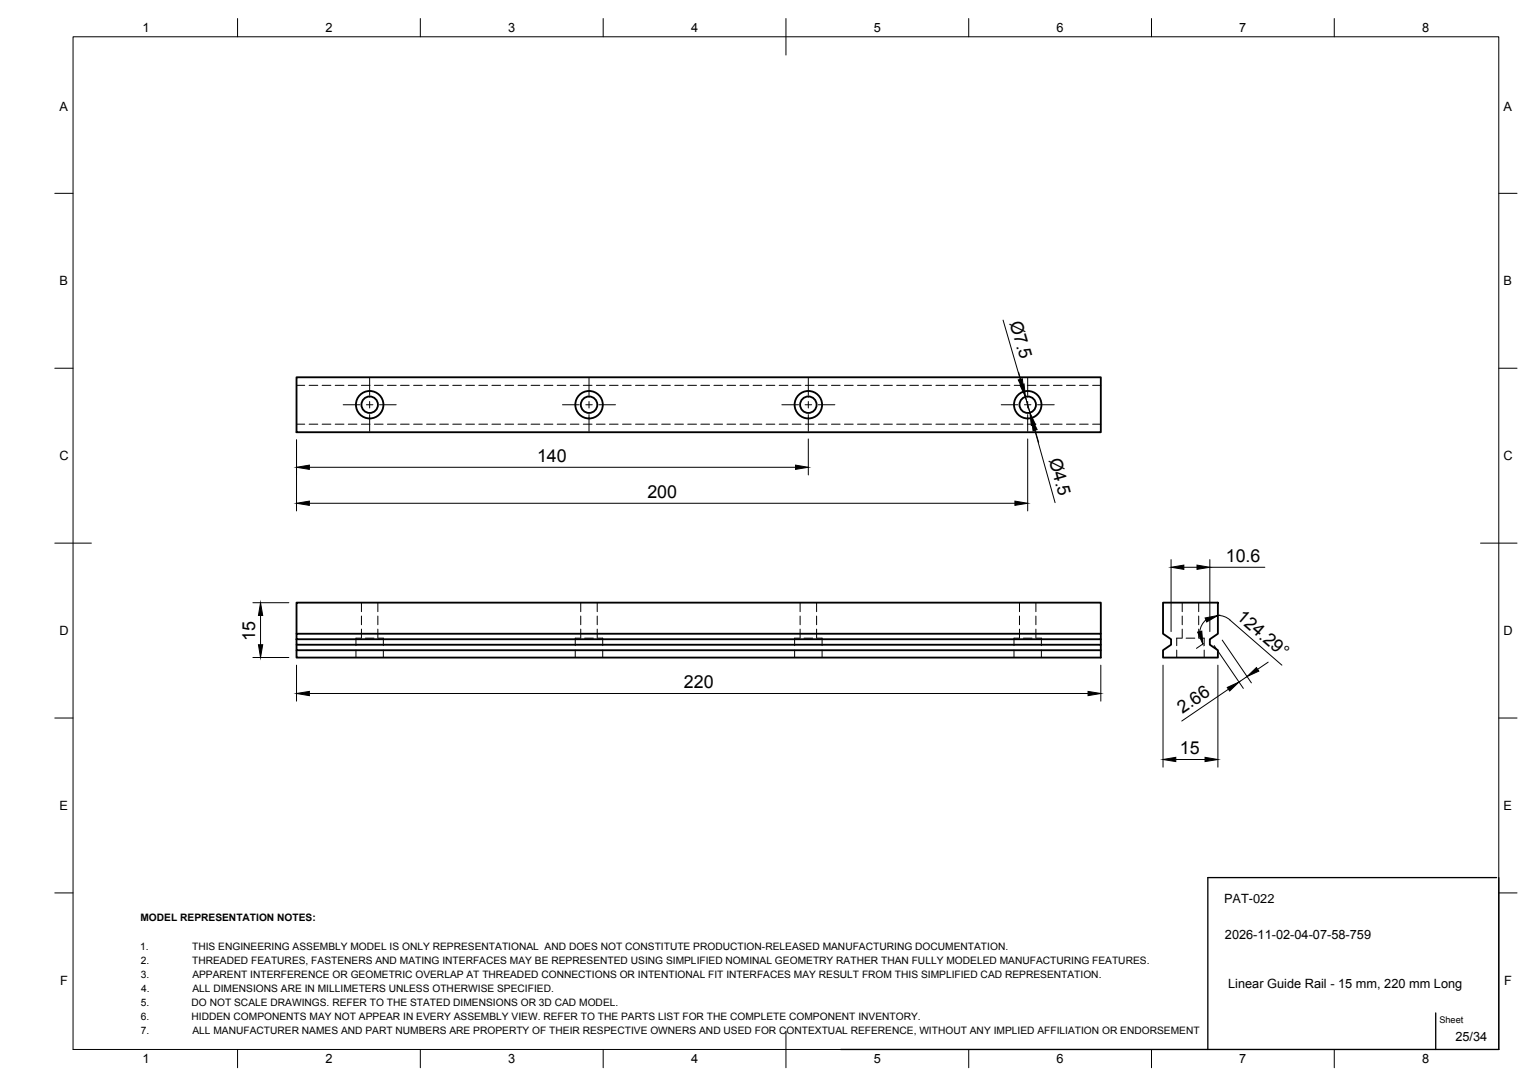
ISO-10303-21;
HEADER;
/* Generated by software containing ST-Developer
 * from STEP Tools, Inc. (www.steptools.com) 
 */

FILE_DESCRIPTION(
/* description */ ('Chute with adjustable gate'),
/* implementation_level */ '2;1');

FILE_NAME(
/* name */ 'Linear Guide Rail - 15 mm, 220 mm Long.step',
/* time_stamp */ '2026-10-27T10:52:28-07:00',
/* author */ (''),
/* organization */ (''),
/* preprocessor_version */ 'ST-DEVELOPER v20.2',
/* originating_system */ 'Autodesk Translation Framework v15.17.0.0',
/* authorisation */ '');

FILE_SCHEMA (('AUTOMOTIVE_DESIGN { 1 0 10303 214 3 1 1 }'));
ENDSEC;

DATA;
#10=MECHANICAL_DESIGN_GEOMETRIC_PRESENTATION_REPRESENTATION('',(#435),#13094);
#371=SHAPE_REPRESENTATION_RELATIONSHIP('SRR','None',#13272,#403);
#403=ADVANCED_BREP_SHAPE_REPRESENTATION('',(#466),#13081);
#435=STYLED_ITEM('',(#13488),#466);
#466=MANIFOLD_SOLID_BREP('Body1',#7619);
#553=FACE_BOUND('',#1658,.T.);
#554=FACE_BOUND('',#1661,.T.);
#555=FACE_BOUND('',#1664,.T.);
#556=FACE_BOUND('',#1667,.T.);
#557=FACE_BOUND('',#1677,.T.);
#558=FACE_BOUND('',#1678,.T.);
#559=FACE_BOUND('',#1679,.T.);
#560=FACE_BOUND('',#1680,.T.);
#561=FACE_BOUND('',#1687,.T.);
#562=FACE_BOUND('',#1688,.T.);
#563=FACE_BOUND('',#1689,.T.);
#564=FACE_BOUND('',#1690,.T.);
#791=PLANE('',#8351);
#792=PLANE('',#8356);
#793=PLANE('',#8361);
#794=PLANE('',#8366);
#795=PLANE('',#8376);
#796=PLANE('',#8377);
#797=PLANE('',#8378);
#798=PLANE('',#8379);
#799=PLANE('',#8380);
#800=PLANE('',#8381);
#801=PLANE('',#8382);
#802=PLANE('',#8383);
#803=PLANE('',#8384);
#804=PLANE('',#8385);
#805=PLANE('',#8386);
#806=PLANE('',#8387);
#807=PLANE('',#8388);
#808=PLANE('',#8389);
#1162=FACE_OUTER_BOUND('',#1656,.T.);
#1163=FACE_OUTER_BOUND('',#1657,.T.);
#1164=FACE_OUTER_BOUND('',#1659,.T.);
#1165=FACE_OUTER_BOUND('',#1660,.T.);
#1166=FACE_OUTER_BOUND('',#1662,.T.);
#1167=FACE_OUTER_BOUND('',#1663,.T.);
#1168=FACE_OUTER_BOUND('',#1665,.T.);
#1169=FACE_OUTER_BOUND('',#1666,.T.);
#1170=FACE_OUTER_BOUND('',#1668,.T.);
#1171=FACE_OUTER_BOUND('',#1669,.T.);
#1172=FACE_OUTER_BOUND('',#1670,.T.);
#1173=FACE_OUTER_BOUND('',#1671,.T.);
#1174=FACE_OUTER_BOUND('',#1672,.T.);
#1175=FACE_OUTER_BOUND('',#1673,.T.);
#1176=FACE_OUTER_BOUND('',#1674,.T.);
#1177=FACE_OUTER_BOUND('',#1675,.T.);
#1178=FACE_OUTER_BOUND('',#1676,.T.);
#1179=FACE_OUTER_BOUND('',#1681,.T.);
#1180=FACE_OUTER_BOUND('',#1682,.T.);
#1181=FACE_OUTER_BOUND('',#1683,.T.);
#1182=FACE_OUTER_BOUND('',#1684,.T.);
#1183=FACE_OUTER_BOUND('',#1685,.T.);
#1184=FACE_OUTER_BOUND('',#1686,.T.);
#1185=FACE_OUTER_BOUND('',#1691,.T.);
#1186=FACE_OUTER_BOUND('',#1692,.T.);
#1187=FACE_OUTER_BOUND('',#1693,.T.);
#1656=EDGE_LOOP('',(#6336,#6337,#6338,#6339));
#1657=EDGE_LOOP('',(#6340));
#1658=EDGE_LOOP('',(#6341));
#1659=EDGE_LOOP('',(#6342,#6343,#6344,#6345));
#1660=EDGE_LOOP('',(#6346));
#1661=EDGE_LOOP('',(#6347));
#1662=EDGE_LOOP('',(#6348,#6349,#6350,#6351));
#1663=EDGE_LOOP('',(#6352));
#1664=EDGE_LOOP('',(#6353));
#1665=EDGE_LOOP('',(#6354,#6355,#6356,#6357));
#1666=EDGE_LOOP('',(#6358));
#1667=EDGE_LOOP('',(#6359));
#1668=EDGE_LOOP('',(#6360,#6361,#6362,#6363));
#1669=EDGE_LOOP('',(#6364,#6365,#6366,#6367));
#1670=EDGE_LOOP('',(#6368,#6369,#6370,#6371));
#1671=EDGE_LOOP('',(#6372,#6373,#6374,#6375));
#1672=EDGE_LOOP('',(#6376,#6377,#6378,#6379));
#1673=EDGE_LOOP('',(#6380,#6381,#6382,#6383));
#1674=EDGE_LOOP('',(#6384,#6385,#6386,#6387));
#1675=EDGE_LOOP('',(#6388,#6389,#6390,#6391));
#1676=EDGE_LOOP('',(#6392,#6393,#6394,#6395));
#1677=EDGE_LOOP('',(#6396));
#1678=EDGE_LOOP('',(#6397));
#1679=EDGE_LOOP('',(#6398));
#1680=EDGE_LOOP('',(#6399));
#1681=EDGE_LOOP('',(#6400,#6401,#6402,#6403));
#1682=EDGE_LOOP('',(#6404,#6405,#6406,#6407));
#1683=EDGE_LOOP('',(#6408,#6409,#6410,#6411));
#1684=EDGE_LOOP('',(#6412,#6413,#6414,#6415));
#1685=EDGE_LOOP('',(#6416,#6417,#6418,#6419));
#1686=EDGE_LOOP('',(#6420,#6421,#6422,#6423));
#1687=EDGE_LOOP('',(#6424));
#1688=EDGE_LOOP('',(#6425));
#1689=EDGE_LOOP('',(#6426));
#1690=EDGE_LOOP('',(#6427));
#1691=EDGE_LOOP('',(#6428,#6429,#6430,#6431));
#1692=EDGE_LOOP('',(#6432,#6433,#6434,#6435,#6436,#6437,#6438,#6439,#6440,
#6441,#6442,#6443));
#1693=EDGE_LOOP('',(#6444,#6445,#6446,#6447,#6448,#6449,#6450,#6451,#6452,
#6453,#6454,#6455));
#2345=LINE('',#12132,#3122);
#2346=LINE('',#12141,#3123);
#2347=LINE('',#12150,#3124);
#2348=LINE('',#12159,#3125);
#2349=LINE('',#12167,#3126);
#2350=LINE('',#12171,#3127);
#2351=LINE('',#12175,#3128);
#2352=LINE('',#12179,#3129);
#2353=LINE('',#12183,#3130);
#2354=LINE('',#12185,#3131);
#2355=LINE('',#12187,#3132);
#2356=LINE('',#12188,#3133);
#2357=LINE('',#12191,#3134);
#2358=LINE('',#12193,#3135);
#2359=LINE('',#12194,#3136);
#2360=LINE('',#12197,#3137);
#2361=LINE('',#12199,#3138);
#2362=LINE('',#12200,#3139);
#2363=LINE('',#12203,#3140);
#2364=LINE('',#12205,#3141);
#2365=LINE('',#12206,#3142);
#2366=LINE('',#12209,#3143);
#2367=LINE('',#12211,#3144);
#2368=LINE('',#12212,#3145);
#2369=LINE('',#12215,#3146);
#2370=LINE('',#12217,#3147);
#2371=LINE('',#12218,#3148);
#2372=LINE('',#12221,#3149);
#2373=LINE('',#12223,#3150);
#2374=LINE('',#12224,#3151);
#2375=LINE('',#12227,#3152);
#2376=LINE('',#12229,#3153);
#2377=LINE('',#12230,#3154);
#2378=LINE('',#12233,#3155);
#2379=LINE('',#12235,#3156);
#2380=LINE('',#12236,#3157);
#2381=LINE('',#12239,#3158);
#2382=LINE('',#12241,#3159);
#2383=LINE('',#12242,#3160);
#2384=LINE('',#12245,#3161);
#2385=LINE('',#12247,#3162);
#2386=LINE('',#12248,#3163);
#2387=LINE('',#12250,#3164);
#2388=LINE('',#12251,#3165);
#3122=VECTOR('',#9911,0.375);
#3123=VECTOR('',#9922,0.375);
#3124=VECTOR('',#9933,0.375);
#3125=VECTOR('',#9944,0.375);
#3126=VECTOR('',#9955,0.225);
#3127=VECTOR('',#9960,0.225);
#3128=VECTOR('',#9965,0.225);
#3129=VECTOR('',#9970,0.225000000000001);
#3130=VECTOR('',#9973,1.);
#3131=VECTOR('',#9974,1.);
#3132=VECTOR('',#9975,1.);
#3133=VECTOR('',#9976,1.);
#3134=VECTOR('',#9979,1.);
#3135=VECTOR('',#9980,1.);
#3136=VECTOR('',#9981,1.);
#3137=VECTOR('',#9984,1.);
#3138=VECTOR('',#9985,1.);
#3139=VECTOR('',#9986,1.);
#3140=VECTOR('',#9989,1.);
#3141=VECTOR('',#9990,1.);
#3142=VECTOR('',#9991,1.);
#3143=VECTOR('',#9994,1.);
#3144=VECTOR('',#9995,1.);
#3145=VECTOR('',#9996,1.);
#3146=VECTOR('',#9999,1.);
#3147=VECTOR('',#10000,1.);
#3148=VECTOR('',#10001,1.);
#3149=VECTOR('',#10004,1.);
#3150=VECTOR('',#10005,1.);
#3151=VECTOR('',#10006,1.);
#3152=VECTOR('',#10009,1.);
#3153=VECTOR('',#10010,1.);
#3154=VECTOR('',#10011,1.);
#3155=VECTOR('',#10014,1.);
#3156=VECTOR('',#10015,1.);
#3157=VECTOR('',#10016,1.);
#3158=VECTOR('',#10019,1.);
#3159=VECTOR('',#10020,1.);
#3160=VECTOR('',#10021,1.);
#3161=VECTOR('',#10024,1.);
#3162=VECTOR('',#10025,1.);
#3163=VECTOR('',#10026,1.);
#3164=VECTOR('',#10029,1.);
#3165=VECTOR('',#10030,1.);
#3504=CIRCLE('',#8349,0.375);
#3505=CIRCLE('',#8350,0.375);
#3506=CIRCLE('',#8352,0.225);
#3507=CIRCLE('',#8354,0.375);
#3508=CIRCLE('',#8355,0.375);
#3509=CIRCLE('',#8357,0.225);
#3510=CIRCLE('',#8359,0.375);
#3511=CIRCLE('',#8360,0.375);
#3512=CIRCLE('',#8362,0.225);
#3513=CIRCLE('',#8364,0.375);
#3514=CIRCLE('',#8365,0.375);
#3515=CIRCLE('',#8367,0.225000000000001);
#3516=CIRCLE('',#8369,0.225);
#3517=CIRCLE('',#8371,0.225);
#3518=CIRCLE('',#8373,0.225);
#3519=CIRCLE('',#8375,0.225000000000001);
#3975=VERTEX_POINT('',#12129);
#3976=VERTEX_POINT('',#12131);
#3977=VERTEX_POINT('',#12135);
#3978=VERTEX_POINT('',#12138);
#3979=VERTEX_POINT('',#12140);
#3980=VERTEX_POINT('',#12144);
#3981=VERTEX_POINT('',#12147);
#3982=VERTEX_POINT('',#12149);
#3983=VERTEX_POINT('',#12153);
#3984=VERTEX_POINT('',#12156);
#3985=VERTEX_POINT('',#12158);
#3986=VERTEX_POINT('',#12162);
#3987=VERTEX_POINT('',#12165);
#3988=VERTEX_POINT('',#12169);
#3989=VERTEX_POINT('',#12173);
#3990=VERTEX_POINT('',#12177);
#3991=VERTEX_POINT('',#12181);
#3992=VERTEX_POINT('',#12182);
#3993=VERTEX_POINT('',#12184);
#3994=VERTEX_POINT('',#12186);
#3995=VERTEX_POINT('',#12190);
#3996=VERTEX_POINT('',#12192);
#3997=VERTEX_POINT('',#12196);
#3998=VERTEX_POINT('',#12198);
#3999=VERTEX_POINT('',#12202);
#4000=VERTEX_POINT('',#12204);
#4001=VERTEX_POINT('',#12208);
#4002=VERTEX_POINT('',#12210);
#4003=VERTEX_POINT('',#12214);
#4004=VERTEX_POINT('',#12216);
#4005=VERTEX_POINT('',#12220);
#4006=VERTEX_POINT('',#12222);
#4007=VERTEX_POINT('',#12226);
#4008=VERTEX_POINT('',#12228);
#4009=VERTEX_POINT('',#12232);
#4010=VERTEX_POINT('',#12234);
#4011=VERTEX_POINT('',#12238);
#4012=VERTEX_POINT('',#12240);
#4013=VERTEX_POINT('',#12244);
#4014=VERTEX_POINT('',#12246);
#4801=EDGE_CURVE('',#3975,#3975,#3504,.T.);
#4802=EDGE_CURVE('',#3975,#3976,#2345,.T.);
#4803=EDGE_CURVE('',#3976,#3976,#3505,.T.);
#4804=EDGE_CURVE('',#3977,#3977,#3506,.T.);
#4805=EDGE_CURVE('',#3978,#3978,#3507,.T.);
#4806=EDGE_CURVE('',#3978,#3979,#2346,.T.);
#4807=EDGE_CURVE('',#3979,#3979,#3508,.T.);
#4808=EDGE_CURVE('',#3980,#3980,#3509,.T.);
#4809=EDGE_CURVE('',#3981,#3981,#3510,.T.);
#4810=EDGE_CURVE('',#3981,#3982,#2347,.T.);
#4811=EDGE_CURVE('',#3982,#3982,#3511,.T.);
#4812=EDGE_CURVE('',#3983,#3983,#3512,.T.);
#4813=EDGE_CURVE('',#3984,#3984,#3513,.T.);
#4814=EDGE_CURVE('',#3984,#3985,#2348,.T.);
#4815=EDGE_CURVE('',#3985,#3985,#3514,.T.);
#4816=EDGE_CURVE('',#3986,#3986,#3515,.T.);
#4817=EDGE_CURVE('',#3987,#3987,#3516,.T.);
#4818=EDGE_CURVE('',#3987,#3977,#2349,.T.);
#4819=EDGE_CURVE('',#3988,#3988,#3517,.T.);
#4820=EDGE_CURVE('',#3988,#3980,#2350,.T.);
#4821=EDGE_CURVE('',#3989,#3989,#3518,.T.);
#4822=EDGE_CURVE('',#3989,#3983,#2351,.T.);
#4823=EDGE_CURVE('',#3990,#3990,#3519,.T.);
#4824=EDGE_CURVE('',#3990,#3986,#2352,.T.);
#4825=EDGE_CURVE('',#3991,#3992,#2353,.T.);
#4826=EDGE_CURVE('',#3992,#3993,#2354,.T.);
#4827=EDGE_CURVE('',#3994,#3993,#2355,.T.);
#4828=EDGE_CURVE('',#3991,#3994,#2356,.T.);
#4829=EDGE_CURVE('',#3995,#3991,#2357,.T.);
#4830=EDGE_CURVE('',#3996,#3994,#2358,.T.);
#4831=EDGE_CURVE('',#3995,#3996,#2359,.T.);
#4832=EDGE_CURVE('',#3997,#3995,#2360,.T.);
#4833=EDGE_CURVE('',#3998,#3996,#2361,.T.);
#4834=EDGE_CURVE('',#3997,#3998,#2362,.T.);
#4835=EDGE_CURVE('',#3999,#3997,#2363,.T.);
#4836=EDGE_CURVE('',#4000,#3998,#2364,.T.);
#4837=EDGE_CURVE('',#3999,#4000,#2365,.T.);
#4838=EDGE_CURVE('',#4001,#3999,#2366,.T.);
#4839=EDGE_CURVE('',#4002,#4000,#2367,.T.);
#4840=EDGE_CURVE('',#4001,#4002,#2368,.T.);
#4841=EDGE_CURVE('',#4003,#4001,#2369,.T.);
#4842=EDGE_CURVE('',#4004,#4002,#2370,.T.);
#4843=EDGE_CURVE('',#4003,#4004,#2371,.T.);
#4844=EDGE_CURVE('',#4005,#4003,#2372,.T.);
#4845=EDGE_CURVE('',#4006,#4004,#2373,.T.);
#4846=EDGE_CURVE('',#4005,#4006,#2374,.T.);
#4847=EDGE_CURVE('',#4007,#4005,#2375,.T.);
#4848=EDGE_CURVE('',#4008,#4006,#2376,.T.);
#4849=EDGE_CURVE('',#4007,#4008,#2377,.T.);
#4850=EDGE_CURVE('',#4009,#4007,#2378,.T.);
#4851=EDGE_CURVE('',#4010,#4008,#2379,.T.);
#4852=EDGE_CURVE('',#4009,#4010,#2380,.T.);
#4853=EDGE_CURVE('',#4011,#4009,#2381,.T.);
#4854=EDGE_CURVE('',#4012,#4010,#2382,.T.);
#4855=EDGE_CURVE('',#4011,#4012,#2383,.T.);
#4856=EDGE_CURVE('',#4013,#4011,#2384,.T.);
#4857=EDGE_CURVE('',#4014,#4012,#2385,.T.);
#4858=EDGE_CURVE('',#4013,#4014,#2386,.T.);
#4859=EDGE_CURVE('',#3992,#4013,#2387,.T.);
#4860=EDGE_CURVE('',#3993,#4014,#2388,.T.);
#6336=ORIENTED_EDGE('',*,*,#4801,.F.);
#6337=ORIENTED_EDGE('',*,*,#4802,.T.);
#6338=ORIENTED_EDGE('',*,*,#4803,.F.);
#6339=ORIENTED_EDGE('',*,*,#4802,.F.);
#6340=ORIENTED_EDGE('',*,*,#4801,.T.);
#6341=ORIENTED_EDGE('',*,*,#4804,.F.);
#6342=ORIENTED_EDGE('',*,*,#4805,.F.);
#6343=ORIENTED_EDGE('',*,*,#4806,.T.);
#6344=ORIENTED_EDGE('',*,*,#4807,.F.);
#6345=ORIENTED_EDGE('',*,*,#4806,.F.);
#6346=ORIENTED_EDGE('',*,*,#4805,.T.);
#6347=ORIENTED_EDGE('',*,*,#4808,.F.);
#6348=ORIENTED_EDGE('',*,*,#4809,.F.);
#6349=ORIENTED_EDGE('',*,*,#4810,.T.);
#6350=ORIENTED_EDGE('',*,*,#4811,.F.);
#6351=ORIENTED_EDGE('',*,*,#4810,.F.);
#6352=ORIENTED_EDGE('',*,*,#4809,.T.);
#6353=ORIENTED_EDGE('',*,*,#4812,.F.);
#6354=ORIENTED_EDGE('',*,*,#4813,.F.);
#6355=ORIENTED_EDGE('',*,*,#4814,.T.);
#6356=ORIENTED_EDGE('',*,*,#4815,.F.);
#6357=ORIENTED_EDGE('',*,*,#4814,.F.);
#6358=ORIENTED_EDGE('',*,*,#4813,.T.);
#6359=ORIENTED_EDGE('',*,*,#4816,.F.);
#6360=ORIENTED_EDGE('',*,*,#4817,.F.);
#6361=ORIENTED_EDGE('',*,*,#4818,.T.);
#6362=ORIENTED_EDGE('',*,*,#4804,.T.);
#6363=ORIENTED_EDGE('',*,*,#4818,.F.);
#6364=ORIENTED_EDGE('',*,*,#4819,.F.);
#6365=ORIENTED_EDGE('',*,*,#4820,.T.);
#6366=ORIENTED_EDGE('',*,*,#4808,.T.);
#6367=ORIENTED_EDGE('',*,*,#4820,.F.);
#6368=ORIENTED_EDGE('',*,*,#4821,.F.);
#6369=ORIENTED_EDGE('',*,*,#4822,.T.);
#6370=ORIENTED_EDGE('',*,*,#4812,.T.);
#6371=ORIENTED_EDGE('',*,*,#4822,.F.);
#6372=ORIENTED_EDGE('',*,*,#4823,.F.);
#6373=ORIENTED_EDGE('',*,*,#4824,.T.);
#6374=ORIENTED_EDGE('',*,*,#4816,.T.);
#6375=ORIENTED_EDGE('',*,*,#4824,.F.);
#6376=ORIENTED_EDGE('',*,*,#4825,.T.);
#6377=ORIENTED_EDGE('',*,*,#4826,.T.);
#6378=ORIENTED_EDGE('',*,*,#4827,.F.);
#6379=ORIENTED_EDGE('',*,*,#4828,.F.);
#6380=ORIENTED_EDGE('',*,*,#4829,.T.);
#6381=ORIENTED_EDGE('',*,*,#4828,.T.);
#6382=ORIENTED_EDGE('',*,*,#4830,.F.);
#6383=ORIENTED_EDGE('',*,*,#4831,.F.);
#6384=ORIENTED_EDGE('',*,*,#4832,.T.);
#6385=ORIENTED_EDGE('',*,*,#4831,.T.);
#6386=ORIENTED_EDGE('',*,*,#4833,.F.);
#6387=ORIENTED_EDGE('',*,*,#4834,.F.);
#6388=ORIENTED_EDGE('',*,*,#4835,.T.);
#6389=ORIENTED_EDGE('',*,*,#4834,.T.);
#6390=ORIENTED_EDGE('',*,*,#4836,.F.);
#6391=ORIENTED_EDGE('',*,*,#4837,.F.);
#6392=ORIENTED_EDGE('',*,*,#4838,.T.);
#6393=ORIENTED_EDGE('',*,*,#4837,.T.);
#6394=ORIENTED_EDGE('',*,*,#4839,.F.);
#6395=ORIENTED_EDGE('',*,*,#4840,.F.);
#6396=ORIENTED_EDGE('',*,*,#4815,.T.);
#6397=ORIENTED_EDGE('',*,*,#4811,.T.);
#6398=ORIENTED_EDGE('',*,*,#4807,.T.);
#6399=ORIENTED_EDGE('',*,*,#4803,.T.);
#6400=ORIENTED_EDGE('',*,*,#4841,.T.);
#6401=ORIENTED_EDGE('',*,*,#4840,.T.);
#6402=ORIENTED_EDGE('',*,*,#4842,.F.);
#6403=ORIENTED_EDGE('',*,*,#4843,.F.);
#6404=ORIENTED_EDGE('',*,*,#4844,.T.);
#6405=ORIENTED_EDGE('',*,*,#4843,.T.);
#6406=ORIENTED_EDGE('',*,*,#4845,.F.);
#6407=ORIENTED_EDGE('',*,*,#4846,.F.);
#6408=ORIENTED_EDGE('',*,*,#4847,.T.);
#6409=ORIENTED_EDGE('',*,*,#4846,.T.);
#6410=ORIENTED_EDGE('',*,*,#4848,.F.);
#6411=ORIENTED_EDGE('',*,*,#4849,.F.);
#6412=ORIENTED_EDGE('',*,*,#4850,.T.);
#6413=ORIENTED_EDGE('',*,*,#4849,.T.);
#6414=ORIENTED_EDGE('',*,*,#4851,.F.);
#6415=ORIENTED_EDGE('',*,*,#4852,.F.);
#6416=ORIENTED_EDGE('',*,*,#4853,.T.);
#6417=ORIENTED_EDGE('',*,*,#4852,.T.);
#6418=ORIENTED_EDGE('',*,*,#4854,.F.);
#6419=ORIENTED_EDGE('',*,*,#4855,.F.);
#6420=ORIENTED_EDGE('',*,*,#4856,.T.);
#6421=ORIENTED_EDGE('',*,*,#4855,.T.);
#6422=ORIENTED_EDGE('',*,*,#4857,.F.);
#6423=ORIENTED_EDGE('',*,*,#4858,.F.);
#6424=ORIENTED_EDGE('',*,*,#4817,.T.);
#6425=ORIENTED_EDGE('',*,*,#4819,.T.);
#6426=ORIENTED_EDGE('',*,*,#4821,.T.);
#6427=ORIENTED_EDGE('',*,*,#4823,.T.);
#6428=ORIENTED_EDGE('',*,*,#4859,.T.);
#6429=ORIENTED_EDGE('',*,*,#4858,.T.);
#6430=ORIENTED_EDGE('',*,*,#4860,.F.);
#6431=ORIENTED_EDGE('',*,*,#4826,.F.);
#6432=ORIENTED_EDGE('',*,*,#4860,.T.);
#6433=ORIENTED_EDGE('',*,*,#4857,.T.);
#6434=ORIENTED_EDGE('',*,*,#4854,.T.);
#6435=ORIENTED_EDGE('',*,*,#4851,.T.);
#6436=ORIENTED_EDGE('',*,*,#4848,.T.);
#6437=ORIENTED_EDGE('',*,*,#4845,.T.);
#6438=ORIENTED_EDGE('',*,*,#4842,.T.);
#6439=ORIENTED_EDGE('',*,*,#4839,.T.);
#6440=ORIENTED_EDGE('',*,*,#4836,.T.);
#6441=ORIENTED_EDGE('',*,*,#4833,.T.);
#6442=ORIENTED_EDGE('',*,*,#4830,.T.);
#6443=ORIENTED_EDGE('',*,*,#4827,.T.);
#6444=ORIENTED_EDGE('',*,*,#4859,.F.);
#6445=ORIENTED_EDGE('',*,*,#4825,.F.);
#6446=ORIENTED_EDGE('',*,*,#4829,.F.);
#6447=ORIENTED_EDGE('',*,*,#4832,.F.);
#6448=ORIENTED_EDGE('',*,*,#4835,.F.);
#6449=ORIENTED_EDGE('',*,*,#4838,.F.);
#6450=ORIENTED_EDGE('',*,*,#4841,.F.);
#6451=ORIENTED_EDGE('',*,*,#4844,.F.);
#6452=ORIENTED_EDGE('',*,*,#4847,.F.);
#6453=ORIENTED_EDGE('',*,*,#4850,.F.);
#6454=ORIENTED_EDGE('',*,*,#4853,.F.);
#6455=ORIENTED_EDGE('',*,*,#4856,.F.);
#7149=CYLINDRICAL_SURFACE('',#8348,0.375);
#7150=CYLINDRICAL_SURFACE('',#8353,0.375);
#7151=CYLINDRICAL_SURFACE('',#8358,0.375);
#7152=CYLINDRICAL_SURFACE('',#8363,0.375);
#7153=CYLINDRICAL_SURFACE('',#8368,0.225);
#7154=CYLINDRICAL_SURFACE('',#8370,0.225);
#7155=CYLINDRICAL_SURFACE('',#8372,0.225);
#7156=CYLINDRICAL_SURFACE('',#8374,0.225000000000001);
#7430=ADVANCED_FACE('',(#1162),#7149,.F.);
#7431=ADVANCED_FACE('',(#1163,#553),#791,.T.);
#7432=ADVANCED_FACE('',(#1164),#7150,.F.);
#7433=ADVANCED_FACE('',(#1165,#554),#792,.T.);
#7434=ADVANCED_FACE('',(#1166),#7151,.F.);
#7435=ADVANCED_FACE('',(#1167,#555),#793,.T.);
#7436=ADVANCED_FACE('',(#1168),#7152,.F.);
#7437=ADVANCED_FACE('',(#1169,#556),#794,.T.);
#7438=ADVANCED_FACE('',(#1170),#7153,.F.);
#7439=ADVANCED_FACE('',(#1171),#7154,.F.);
#7440=ADVANCED_FACE('',(#1172),#7155,.F.);
#7441=ADVANCED_FACE('',(#1173),#7156,.F.);
#7442=ADVANCED_FACE('',(#1174),#795,.T.);
#7443=ADVANCED_FACE('',(#1175),#796,.T.);
#7444=ADVANCED_FACE('',(#1176),#797,.T.);
#7445=ADVANCED_FACE('',(#1177),#798,.T.);
#7446=ADVANCED_FACE('',(#1178,#557,#558,#559,#560),#799,.T.);
#7447=ADVANCED_FACE('',(#1179),#800,.T.);
#7448=ADVANCED_FACE('',(#1180),#801,.T.);
#7449=ADVANCED_FACE('',(#1181),#802,.T.);
#7450=ADVANCED_FACE('',(#1182),#803,.T.);
#7451=ADVANCED_FACE('',(#1183),#804,.T.);
#7452=ADVANCED_FACE('',(#1184,#561,#562,#563,#564),#805,.T.);
#7453=ADVANCED_FACE('',(#1185),#806,.T.);
#7454=ADVANCED_FACE('',(#1186),#807,.T.);
#7455=ADVANCED_FACE('',(#1187),#808,.F.);
#7619=CLOSED_SHELL('',(#7430,#7431,#7432,#7433,#7434,#7435,#7436,#7437,
#7438,#7439,#7440,#7441,#7442,#7443,#7444,#7445,#7446,#7447,#7448,#7449,
#7450,#7451,#7452,#7453,#7454,#7455));
#8347=AXIS2_PLACEMENT_3D('',#12127,#9905,#9906);
#8348=AXIS2_PLACEMENT_3D('',#12128,#9907,#9908);
#8349=AXIS2_PLACEMENT_3D('',#12130,#9909,#9910);
#8350=AXIS2_PLACEMENT_3D('',#12133,#9912,#9913);
#8351=AXIS2_PLACEMENT_3D('',#12134,#9914,#9915);
#8352=AXIS2_PLACEMENT_3D('',#12136,#9916,#9917);
#8353=AXIS2_PLACEMENT_3D('',#12137,#9918,#9919);
#8354=AXIS2_PLACEMENT_3D('',#12139,#9920,#9921);
#8355=AXIS2_PLACEMENT_3D('',#12142,#9923,#9924);
#8356=AXIS2_PLACEMENT_3D('',#12143,#9925,#9926);
#8357=AXIS2_PLACEMENT_3D('',#12145,#9927,#9928);
#8358=AXIS2_PLACEMENT_3D('',#12146,#9929,#9930);
#8359=AXIS2_PLACEMENT_3D('',#12148,#9931,#9932);
#8360=AXIS2_PLACEMENT_3D('',#12151,#9934,#9935);
#8361=AXIS2_PLACEMENT_3D('',#12152,#9936,#9937);
#8362=AXIS2_PLACEMENT_3D('',#12154,#9938,#9939);
#8363=AXIS2_PLACEMENT_3D('',#12155,#9940,#9941);
#8364=AXIS2_PLACEMENT_3D('',#12157,#9942,#9943);
#8365=AXIS2_PLACEMENT_3D('',#12160,#9945,#9946);
#8366=AXIS2_PLACEMENT_3D('',#12161,#9947,#9948);
#8367=AXIS2_PLACEMENT_3D('',#12163,#9949,#9950);
#8368=AXIS2_PLACEMENT_3D('',#12164,#9951,#9952);
#8369=AXIS2_PLACEMENT_3D('',#12166,#9953,#9954);
#8370=AXIS2_PLACEMENT_3D('',#12168,#9956,#9957);
#8371=AXIS2_PLACEMENT_3D('',#12170,#9958,#9959);
#8372=AXIS2_PLACEMENT_3D('',#12172,#9961,#9962);
#8373=AXIS2_PLACEMENT_3D('',#12174,#9963,#9964);
#8374=AXIS2_PLACEMENT_3D('',#12176,#9966,#9967);
#8375=AXIS2_PLACEMENT_3D('',#12178,#9968,#9969);
#8376=AXIS2_PLACEMENT_3D('',#12180,#9971,#9972);
#8377=AXIS2_PLACEMENT_3D('',#12189,#9977,#9978);
#8378=AXIS2_PLACEMENT_3D('',#12195,#9982,#9983);
#8379=AXIS2_PLACEMENT_3D('',#12201,#9987,#9988);
#8380=AXIS2_PLACEMENT_3D('',#12207,#9992,#9993);
#8381=AXIS2_PLACEMENT_3D('',#12213,#9997,#9998);
#8382=AXIS2_PLACEMENT_3D('',#12219,#10002,#10003);
#8383=AXIS2_PLACEMENT_3D('',#12225,#10007,#10008);
#8384=AXIS2_PLACEMENT_3D('',#12231,#10012,#10013);
#8385=AXIS2_PLACEMENT_3D('',#12237,#10017,#10018);
#8386=AXIS2_PLACEMENT_3D('',#12243,#10022,#10023);
#8387=AXIS2_PLACEMENT_3D('',#12249,#10027,#10028);
#8388=AXIS2_PLACEMENT_3D('',#12252,#10031,#10032);
#8389=AXIS2_PLACEMENT_3D('',#12253,#10033,#10034);
#9905=DIRECTION('axis',(0.,0.,1.));
#9906=DIRECTION('refdir',(1.,0.,0.));
#9907=DIRECTION('center_axis',(0.,0.,1.));
#9908=DIRECTION('ref_axis',(1.,0.,0.));
#9909=DIRECTION('center_axis',(0.,0.,1.));
#9910=DIRECTION('ref_axis',(1.,0.,0.));
#9911=DIRECTION('',(0.,0.,1.));
#9912=DIRECTION('center_axis',(0.,0.,-1.));
#9913=DIRECTION('ref_axis',(1.,0.,0.));
#9914=DIRECTION('center_axis',(0.,0.,1.));
#9915=DIRECTION('ref_axis',(1.,0.,0.));
#9916=DIRECTION('center_axis',(0.,0.,1.));
#9917=DIRECTION('ref_axis',(1.,0.,0.));
#9918=DIRECTION('center_axis',(0.,0.,1.));
#9919=DIRECTION('ref_axis',(1.,0.,0.));
#9920=DIRECTION('center_axis',(0.,0.,1.));
#9921=DIRECTION('ref_axis',(1.,0.,0.));
#9922=DIRECTION('',(0.,0.,1.));
#9923=DIRECTION('center_axis',(0.,0.,-1.));
#9924=DIRECTION('ref_axis',(1.,0.,0.));
#9925=DIRECTION('center_axis',(0.,0.,1.));
#9926=DIRECTION('ref_axis',(1.,0.,0.));
#9927=DIRECTION('center_axis',(0.,0.,1.));
#9928=DIRECTION('ref_axis',(1.,0.,0.));
#9929=DIRECTION('center_axis',(0.,0.,1.));
#9930=DIRECTION('ref_axis',(1.,0.,0.));
#9931=DIRECTION('center_axis',(0.,0.,1.));
#9932=DIRECTION('ref_axis',(1.,0.,0.));
#9933=DIRECTION('',(0.,0.,1.));
#9934=DIRECTION('center_axis',(0.,0.,-1.));
#9935=DIRECTION('ref_axis',(1.,0.,0.));
#9936=DIRECTION('center_axis',(0.,0.,1.));
#9937=DIRECTION('ref_axis',(1.,0.,0.));
#9938=DIRECTION('center_axis',(0.,0.,1.));
#9939=DIRECTION('ref_axis',(1.,0.,0.));
#9940=DIRECTION('center_axis',(0.,0.,1.));
#9941=DIRECTION('ref_axis',(1.,0.,0.));
#9942=DIRECTION('center_axis',(0.,0.,1.));
#9943=DIRECTION('ref_axis',(1.,0.,0.));
#9944=DIRECTION('',(0.,0.,1.));
#9945=DIRECTION('center_axis',(0.,0.,-1.));
#9946=DIRECTION('ref_axis',(1.,0.,0.));
#9947=DIRECTION('center_axis',(0.,0.,1.));
#9948=DIRECTION('ref_axis',(1.,0.,0.));
#9949=DIRECTION('center_axis',(0.,0.,1.));
#9950=DIRECTION('ref_axis',(1.,0.,0.));
#9951=DIRECTION('center_axis',(0.,0.,1.));
#9952=DIRECTION('ref_axis',(1.,0.,0.));
#9953=DIRECTION('center_axis',(0.,0.,1.));
#9954=DIRECTION('ref_axis',(1.,0.,0.));
#9955=DIRECTION('',(0.,0.,1.));
#9956=DIRECTION('center_axis',(0.,0.,1.));
#9957=DIRECTION('ref_axis',(1.,0.,0.));
#9958=DIRECTION('center_axis',(0.,0.,1.));
#9959=DIRECTION('ref_axis',(1.,0.,0.));
#9960=DIRECTION('',(0.,0.,1.));
#9961=DIRECTION('center_axis',(0.,0.,1.));
#9962=DIRECTION('ref_axis',(1.,0.,0.));
#9963=DIRECTION('center_axis',(0.,0.,1.));
#9964=DIRECTION('ref_axis',(1.,0.,0.));
#9965=DIRECTION('',(0.,0.,1.));
#9966=DIRECTION('center_axis',(0.,0.,1.));
#9967=DIRECTION('ref_axis',(1.,0.,0.));
#9968=DIRECTION('center_axis',(0.,0.,1.));
#9969=DIRECTION('ref_axis',(1.,0.,0.));
#9970=DIRECTION('',(0.,0.,1.));
#9971=DIRECTION('center_axis',(0.,-0.56333682464151,0.826227342807548));
#9972=DIRECTION('ref_axis',(0.,-0.826227342807548,-0.56333682464151));
#9973=DIRECTION('',(0.,-0.826227342807548,-0.56333682464151));
#9974=DIRECTION('',(1.,0.,0.));
#9975=DIRECTION('',(0.,-0.826227342807548,-0.56333682464151));
#9976=DIRECTION('',(1.,0.,0.));
#9977=DIRECTION('center_axis',(0.,-1.,0.));
#9978=DIRECTION('ref_axis',(0.,0.,-1.));
#9979=DIRECTION('',(0.,0.,-1.));
#9980=DIRECTION('',(0.,0.,-1.));
#9981=DIRECTION('',(1.,0.,0.));
#9982=DIRECTION('center_axis',(0.,-0.56333682464151,-0.826227342807548));
#9983=DIRECTION('ref_axis',(0.,0.826227342807548,-0.56333682464151));
#9984=DIRECTION('',(0.,0.826227342807548,-0.56333682464151));
#9985=DIRECTION('',(0.,0.826227342807548,-0.56333682464151));
#9986=DIRECTION('',(1.,0.,0.));
#9987=DIRECTION('center_axis',(0.,-1.,0.));
#9988=DIRECTION('ref_axis',(0.,0.,-1.));
#9989=DIRECTION('',(0.,0.,-1.));
#9990=DIRECTION('',(0.,0.,-1.));
#9991=DIRECTION('',(1.,0.,0.));
#9992=DIRECTION('center_axis',(0.,0.,1.));
#9993=DIRECTION('ref_axis',(0.,-1.,0.));
#9994=DIRECTION('',(0.,-1.,0.));
#9995=DIRECTION('',(0.,-1.,0.));
#9996=DIRECTION('',(1.,0.,0.));
#9997=DIRECTION('center_axis',(0.,1.,0.));
#9998=DIRECTION('ref_axis',(0.,0.,1.));
#9999=DIRECTION('',(0.,0.,1.));
#10000=DIRECTION('',(0.,0.,1.));
#10001=DIRECTION('',(1.,0.,0.));
#10002=DIRECTION('center_axis',(0.,0.56333682464151,-0.826227342807548));
#10003=DIRECTION('ref_axis',(0.,0.826227342807548,0.56333682464151));
#10004=DIRECTION('',(0.,0.826227342807548,0.56333682464151));
#10005=DIRECTION('',(0.,0.826227342807548,0.56333682464151));
#10006=DIRECTION('',(1.,0.,0.));
#10007=DIRECTION('center_axis',(0.,1.,0.));
#10008=DIRECTION('ref_axis',(0.,0.,1.));
#10009=DIRECTION('',(0.,0.,1.));
#10010=DIRECTION('',(0.,0.,1.));
#10011=DIRECTION('',(1.,0.,0.));
#10012=DIRECTION('center_axis',(0.,0.56333682464151,0.826227342807548));
#10013=DIRECTION('ref_axis',(0.,-0.826227342807548,0.56333682464151));
#10014=DIRECTION('',(0.,-0.826227342807548,0.56333682464151));
#10015=DIRECTION('',(0.,-0.826227342807548,0.56333682464151));
#10016=DIRECTION('',(1.,0.,0.));
#10017=DIRECTION('center_axis',(0.,1.,0.));
#10018=DIRECTION('ref_axis',(0.,0.,1.));
#10019=DIRECTION('',(0.,0.,1.));
#10020=DIRECTION('',(0.,0.,1.));
#10021=DIRECTION('',(1.,0.,0.));
#10022=DIRECTION('center_axis',(0.,0.,-1.));
#10023=DIRECTION('ref_axis',(0.,1.,0.));
#10024=DIRECTION('',(0.,1.,0.));
#10025=DIRECTION('',(0.,1.,0.));
#10026=DIRECTION('',(1.,0.,0.));
#10027=DIRECTION('center_axis',(0.,-1.,0.));
#10028=DIRECTION('ref_axis',(0.,0.,-1.));
#10029=DIRECTION('',(0.,0.,-1.));
#10030=DIRECTION('',(0.,0.,-1.));
#10031=DIRECTION('center_axis',(1.,0.,0.));
#10032=DIRECTION('ref_axis',(0.,0.,-1.));
#10033=DIRECTION('center_axis',(1.,0.,0.));
#10034=DIRECTION('ref_axis',(0.,0.,-1.));
#12127=CARTESIAN_POINT('',(0.,0.,0.));
#12128=CARTESIAN_POINT('Origin',(14.,0.,0.97));
#12129=CARTESIAN_POINT('',(13.625,-4.59242549680257E-17,0.97));
#12130=CARTESIAN_POINT('Origin',(14.,0.,0.97));
#12131=CARTESIAN_POINT('',(13.625,4.59242549680257E-17,1.5));
#12132=CARTESIAN_POINT('',(13.625,-4.59242549680257E-17,0.97));
#12133=CARTESIAN_POINT('Origin',(14.,0.,1.5));
#12134=CARTESIAN_POINT('Origin',(14.,0.,0.97));
#12135=CARTESIAN_POINT('',(13.775,-2.75545529808154E-17,0.97));
#12136=CARTESIAN_POINT('Origin',(14.,0.,0.97));
#12137=CARTESIAN_POINT('Origin',(8.,0.,0.97));
#12138=CARTESIAN_POINT('',(7.625,-4.59242549680257E-17,0.97));
#12139=CARTESIAN_POINT('Origin',(8.,0.,0.97));
#12140=CARTESIAN_POINT('',(7.625,4.59242549680257E-17,1.5));
#12141=CARTESIAN_POINT('',(7.625,-4.59242549680257E-17,0.97));
#12142=CARTESIAN_POINT('Origin',(8.,0.,1.5));
#12143=CARTESIAN_POINT('Origin',(8.,0.,0.97));
#12144=CARTESIAN_POINT('',(7.775,-2.75545529808154E-17,0.97));
#12145=CARTESIAN_POINT('Origin',(8.,0.,0.97));
#12146=CARTESIAN_POINT('Origin',(2.,0.,0.97));
#12147=CARTESIAN_POINT('',(1.625,-4.59242549680257E-17,0.97));
#12148=CARTESIAN_POINT('Origin',(2.,0.,0.97));
#12149=CARTESIAN_POINT('',(1.625,4.59242549680257E-17,1.5));
#12150=CARTESIAN_POINT('',(1.625,-4.59242549680257E-17,0.97));
#12151=CARTESIAN_POINT('Origin',(2.,0.,1.5));
#12152=CARTESIAN_POINT('Origin',(2.,0.,0.97));
#12153=CARTESIAN_POINT('',(1.775,-2.75545529808155E-17,0.97));
#12154=CARTESIAN_POINT('Origin',(2.,0.,0.97));
#12155=CARTESIAN_POINT('Origin',(20.,0.,0.97));
#12156=CARTESIAN_POINT('',(19.625,-4.59242549680257E-17,0.97));
#12157=CARTESIAN_POINT('Origin',(20.,0.,0.97));
#12158=CARTESIAN_POINT('',(19.625,4.59242549680257E-17,1.5));
#12159=CARTESIAN_POINT('',(19.625,-4.59242549680257E-17,0.97));
#12160=CARTESIAN_POINT('Origin',(20.,0.,1.5));
#12161=CARTESIAN_POINT('Origin',(20.,0.,0.97));
#12162=CARTESIAN_POINT('',(19.775,-2.75545529808156E-17,0.97));
#12163=CARTESIAN_POINT('Origin',(20.,0.,0.97));
#12164=CARTESIAN_POINT('Origin',(14.,0.,-0.1));
#12165=CARTESIAN_POINT('',(13.775,-2.75545529808154E-17,0.));
#12166=CARTESIAN_POINT('Origin',(14.,0.,0.));
#12167=CARTESIAN_POINT('',(13.775,-2.75545529808154E-17,-0.1));
#12168=CARTESIAN_POINT('Origin',(8.,0.,-0.1));
#12169=CARTESIAN_POINT('',(7.775,-2.75545529808154E-17,0.));
#12170=CARTESIAN_POINT('Origin',(8.,0.,0.));
#12171=CARTESIAN_POINT('',(7.775,-2.75545529808154E-17,-0.1));
#12172=CARTESIAN_POINT('Origin',(2.,0.,-0.1));
#12173=CARTESIAN_POINT('',(1.775,-2.75545529808155E-17,0.));
#12174=CARTESIAN_POINT('Origin',(2.,0.,0.));
#12175=CARTESIAN_POINT('',(1.775,-2.75545529808155E-17,-0.1));
#12176=CARTESIAN_POINT('Origin',(20.,0.,-0.1));
#12177=CARTESIAN_POINT('',(19.775,-2.75545529808156E-17,0.));
#12178=CARTESIAN_POINT('Origin',(20.,0.,0.));
#12179=CARTESIAN_POINT('',(19.775,-2.75545529808156E-17,-0.1));
#12180=CARTESIAN_POINT('Origin',(0.,-0.53,1.));
#12181=CARTESIAN_POINT('',(0.,-0.53,1.));
#12182=CARTESIAN_POINT('',(0.,-0.75,0.85));
#12183=CARTESIAN_POINT('',(0.,-0.53,1.));
#12184=CARTESIAN_POINT('',(22.,-0.75,0.85));
#12185=CARTESIAN_POINT('',(0.,-0.75,0.85));
#12186=CARTESIAN_POINT('',(22.,-0.53,1.));
#12187=CARTESIAN_POINT('',(22.,-0.53,1.));
#12188=CARTESIAN_POINT('',(0.,-0.53,1.));
#12189=CARTESIAN_POINT('Origin',(0.,-0.53,1.15));
#12190=CARTESIAN_POINT('',(0.,-0.53,1.15));
#12191=CARTESIAN_POINT('',(0.,-0.53,1.15));
#12192=CARTESIAN_POINT('',(22.,-0.53,1.15));
#12193=CARTESIAN_POINT('',(22.,-0.53,1.15));
#12194=CARTESIAN_POINT('',(0.,-0.53,1.15));
#12195=CARTESIAN_POINT('Origin',(0.,-0.75,1.3));
#12196=CARTESIAN_POINT('',(0.,-0.75,1.3));
#12197=CARTESIAN_POINT('',(0.,-0.75,1.3));
#12198=CARTESIAN_POINT('',(22.,-0.75,1.3));
#12199=CARTESIAN_POINT('',(22.,-0.75,1.3));
#12200=CARTESIAN_POINT('',(0.,-0.75,1.3));
#12201=CARTESIAN_POINT('Origin',(0.,-0.75,1.5));
#12202=CARTESIAN_POINT('',(0.,-0.75,1.5));
#12203=CARTESIAN_POINT('',(0.,-0.75,1.5));
#12204=CARTESIAN_POINT('',(22.,-0.75,1.5));
#12205=CARTESIAN_POINT('',(22.,-0.75,1.5));
#12206=CARTESIAN_POINT('',(0.,-0.75,1.5));
#12207=CARTESIAN_POINT('Origin',(0.,0.75,1.5));
#12208=CARTESIAN_POINT('',(0.,0.75,1.5));
#12209=CARTESIAN_POINT('',(0.,0.75,1.5));
#12210=CARTESIAN_POINT('',(22.,0.75,1.5));
#12211=CARTESIAN_POINT('',(22.,0.75,1.5));
#12212=CARTESIAN_POINT('',(0.,0.75,1.5));
#12213=CARTESIAN_POINT('Origin',(0.,0.75,1.3));
#12214=CARTESIAN_POINT('',(0.,0.75,1.3));
#12215=CARTESIAN_POINT('',(0.,0.75,1.3));
#12216=CARTESIAN_POINT('',(22.,0.75,1.3));
#12217=CARTESIAN_POINT('',(22.,0.75,1.3));
#12218=CARTESIAN_POINT('',(0.,0.75,1.3));
#12219=CARTESIAN_POINT('Origin',(0.,0.53,1.15));
#12220=CARTESIAN_POINT('',(0.,0.53,1.15));
#12221=CARTESIAN_POINT('',(0.,0.53,1.15));
#12222=CARTESIAN_POINT('',(22.,0.53,1.15));
#12223=CARTESIAN_POINT('',(22.,0.53,1.15));
#12224=CARTESIAN_POINT('',(0.,0.53,1.15));
#12225=CARTESIAN_POINT('Origin',(0.,0.53,1.));
#12226=CARTESIAN_POINT('',(0.,0.53,1.));
#12227=CARTESIAN_POINT('',(0.,0.53,1.));
#12228=CARTESIAN_POINT('',(22.,0.53,1.));
#12229=CARTESIAN_POINT('',(22.,0.53,1.));
#12230=CARTESIAN_POINT('',(0.,0.53,1.));
#12231=CARTESIAN_POINT('Origin',(0.,0.75,0.85));
#12232=CARTESIAN_POINT('',(0.,0.75,0.85));
#12233=CARTESIAN_POINT('',(0.,0.75,0.85));
#12234=CARTESIAN_POINT('',(22.,0.75,0.85));
#12235=CARTESIAN_POINT('',(22.,0.75,0.85));
#12236=CARTESIAN_POINT('',(0.,0.75,0.85));
#12237=CARTESIAN_POINT('Origin',(0.,0.75,0.));
#12238=CARTESIAN_POINT('',(0.,0.75,0.));
#12239=CARTESIAN_POINT('',(0.,0.75,0.));
#12240=CARTESIAN_POINT('',(22.,0.75,0.));
#12241=CARTESIAN_POINT('',(22.,0.75,0.));
#12242=CARTESIAN_POINT('',(0.,0.75,0.));
#12243=CARTESIAN_POINT('Origin',(0.,-0.75,0.));
#12244=CARTESIAN_POINT('',(0.,-0.75,0.));
#12245=CARTESIAN_POINT('',(0.,-0.75,0.));
#12246=CARTESIAN_POINT('',(22.,-0.75,0.));
#12247=CARTESIAN_POINT('',(22.,-0.75,0.));
#12248=CARTESIAN_POINT('',(0.,-0.75,0.));
#12249=CARTESIAN_POINT('Origin',(0.,-0.75,0.85));
#12250=CARTESIAN_POINT('',(0.,-0.75,0.85));
#12251=CARTESIAN_POINT('',(22.,-0.75,0.85));
#12252=CARTESIAN_POINT('Origin',(22.,0.,0.75));
#12253=CARTESIAN_POINT('Origin',(0.,0.,0.75));
#13044=UNCERTAINTY_MEASURE_WITH_UNIT(LENGTH_MEASURE(0.001),#13095,
'DISTANCE_ACCURACY_VALUE',
'Maximum model space distance between geometric entities at asserted c
onnectivities');
#13057=UNCERTAINTY_MEASURE_WITH_UNIT(LENGTH_MEASURE(0.001),#13095,
'DISTANCE_ACCURACY_VALUE',
'Maximum model space distance between geometric entities at asserted c
onnectivities');
#13081=(
GEOMETRIC_REPRESENTATION_CONTEXT(3)
GLOBAL_UNCERTAINTY_ASSIGNED_CONTEXT((#13044))
GLOBAL_UNIT_ASSIGNED_CONTEXT((#13095,#13097,#13098))
REPRESENTATION_CONTEXT('','3D')
);
#13094=(
GEOMETRIC_REPRESENTATION_CONTEXT(3)
GLOBAL_UNCERTAINTY_ASSIGNED_CONTEXT((#13057))
GLOBAL_UNIT_ASSIGNED_CONTEXT((#13095,#13097,#13098))
REPRESENTATION_CONTEXT('','3D')
);
#13095=(
LENGTH_UNIT()
NAMED_UNIT(*)
SI_UNIT(.CENTI.,.METRE.)
);
#13097=(
NAMED_UNIT(*)
PLANE_ANGLE_UNIT()
SI_UNIT($,.RADIAN.)
);
#13098=(
NAMED_UNIT(*)
SI_UNIT($,.STERADIAN.)
SOLID_ANGLE_UNIT()
);
#13122=SHAPE_DEFINITION_REPRESENTATION(#13158,#13272);
#13158=PRODUCT_DEFINITION_SHAPE('',$,#13309);
#13272=SHAPE_REPRESENTATION('',(#8347),#13081);
#13285=PRODUCT_DEFINITION_CONTEXT('part definition',#13395,'design');
#13309=PRODUCT_DEFINITION('Linear Guide Rail - 15 mm, 220 mm Long',
'Linear Guide Rail - 15 mm, 220 mm Long',#13345,#13285);
#13345=PRODUCT_DEFINITION_FORMATION('',$,#13420);
#13395=APPLICATION_CONTEXT(
'Core Data for Automotive Mechanical Design Process');
#13396=PRODUCT_CONTEXT('part definition',#13395,'mechanical');
#13420=PRODUCT('Linear Guide Rail - 15 mm, 220 mm Long',
'Linear Guide Rail - 15 mm, 220 mm Long',
'Linear Guide Rail - 15 mm, 220 mm Long',(#13396));
#13482=COLOUR_RGB('Sky Blue',0.24,0.69,0.87);
#13483=FILL_AREA_STYLE_COLOUR('',#13482);
#13484=FILL_AREA_STYLE('',(#13483));
#13485=SURFACE_STYLE_FILL_AREA(#13484);
#13486=SURFACE_SIDE_STYLE('',(#13485));
#13487=SURFACE_STYLE_USAGE(.BOTH.,#13486);
#13488=PRESENTATION_STYLE_ASSIGNMENT((#13487));
ENDSEC;
END-ISO-10303-21;
